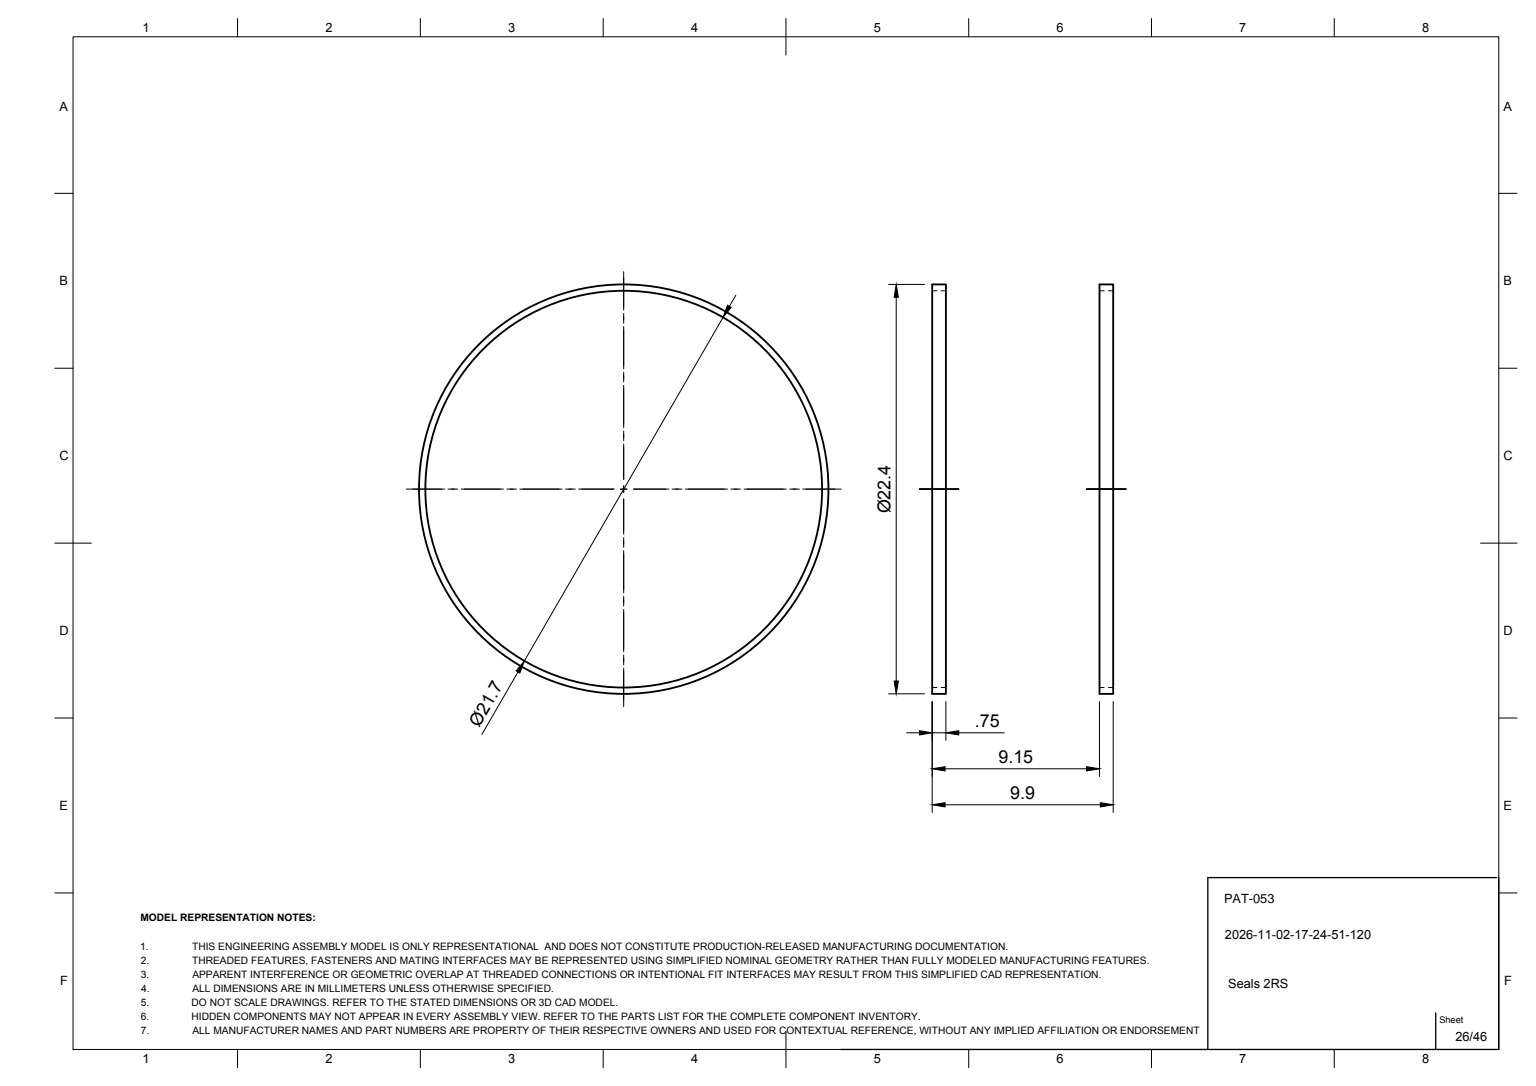
ISO-10303-21;
HEADER;
/* Generated by software containing ST-Developer
 * from STEP Tools, Inc. (www.steptools.com) 
 */

FILE_DESCRIPTION(
/* description */ ('Hand-operated arbor press'),
/* implementation_level */ '2;1');

FILE_NAME(
/* name */ 'Seals 2RS.step',
/* time_stamp */ '2026-10-28T03:25:25-07:00',
/* author */ (''),
/* organization */ (''),
/* preprocessor_version */ 'ST-DEVELOPER v20.2',
/* originating_system */ 'Autodesk Translation Framework v15.17.0.0',
/* authorisation */ '');

FILE_SCHEMA (('AUTOMOTIVE_DESIGN { 1 0 10303 214 3 1 1 }'));
ENDSEC;

DATA;
#10=MECHANICAL_DESIGN_GEOMETRIC_PRESENTATION_REPRESENTATION('',(#612,#613),#32751);
#522=SHAPE_REPRESENTATION_RELATIONSHIP('SRR','None',#32952,#564);
#564=ADVANCED_BREP_SHAPE_REPRESENTATION('',(#660,#661),#32726);
#612=STYLED_ITEM('',(#33242),#660);
#613=STYLED_ITEM('',(#33242),#661);
#660=MANIFOLD_SOLID_BREP('Body1',#12510);
#661=MANIFOLD_SOLID_BREP('Body2',#12511);
#807=FACE_BOUND('',#2361,.T.);
#808=FACE_BOUND('',#2364,.T.);
#809=FACE_BOUND('',#2367,.T.);
#810=FACE_BOUND('',#2370,.T.);
#989=PLANE('',#13521);
#990=PLANE('',#13526);
#991=PLANE('',#13529);
#992=PLANE('',#13534);
#1552=FACE_OUTER_BOUND('',#2360,.T.);
#1553=FACE_OUTER_BOUND('',#2362,.T.);
#1554=FACE_OUTER_BOUND('',#2363,.T.);
#1555=FACE_OUTER_BOUND('',#2365,.T.);
#1556=FACE_OUTER_BOUND('',#2366,.T.);
#1557=FACE_OUTER_BOUND('',#2368,.T.);
#1558=FACE_OUTER_BOUND('',#2369,.T.);
#1559=FACE_OUTER_BOUND('',#2371,.T.);
#2360=EDGE_LOOP('',(#9516));
#2361=EDGE_LOOP('',(#9517));
#2362=EDGE_LOOP('',(#9518,#9519,#9520,#9521));
#2363=EDGE_LOOP('',(#9522));
#2364=EDGE_LOOP('',(#9523));
#2365=EDGE_LOOP('',(#9524,#9525,#9526,#9527));
#2366=EDGE_LOOP('',(#9528));
#2367=EDGE_LOOP('',(#9529));
#2368=EDGE_LOOP('',(#9530,#9531,#9532,#9533));
#2369=EDGE_LOOP('',(#9534));
#2370=EDGE_LOOP('',(#9535));
#2371=EDGE_LOOP('',(#9536,#9537,#9538,#9539));
#3167=LINE('',#19223,#4338);
#3168=LINE('',#19228,#4339);
#3169=LINE('',#19237,#4340);
#3170=LINE('',#19242,#4341);
#4338=VECTOR('',#15552,1.119765);
#4339=VECTOR('',#15559,1.085235);
#4340=VECTOR('',#15570,1.119765);
#4341=VECTOR('',#15577,1.085235);
#5405=CIRCLE('',#13522,1.119765);
#5406=CIRCLE('',#13523,1.085235);
#5407=CIRCLE('',#13525,1.119765);
#5408=CIRCLE('',#13527,1.085235);
#5409=CIRCLE('',#13530,1.119765);
#5410=CIRCLE('',#13531,1.085235);
#5411=CIRCLE('',#13533,1.119765);
#5412=CIRCLE('',#13535,1.085235);
#5960=VERTEX_POINT('',#19216);
#5961=VERTEX_POINT('',#19218);
#5962=VERTEX_POINT('',#19221);
#5963=VERTEX_POINT('',#19225);
#5964=VERTEX_POINT('',#19230);
#5965=VERTEX_POINT('',#19232);
#5966=VERTEX_POINT('',#19235);
#5967=VERTEX_POINT('',#19239);
#7261=EDGE_CURVE('',#5960,#5960,#5405,.T.);
#7262=EDGE_CURVE('',#5961,#5961,#5406,.T.);
#7263=EDGE_CURVE('',#5962,#5962,#5407,.T.);
#7264=EDGE_CURVE('',#5962,#5960,#3167,.T.);
#7265=EDGE_CURVE('',#5963,#5963,#5408,.T.);
#7266=EDGE_CURVE('',#5963,#5961,#3168,.T.);
#7267=EDGE_CURVE('',#5964,#5964,#5409,.T.);
#7268=EDGE_CURVE('',#5965,#5965,#5410,.T.);
#7269=EDGE_CURVE('',#5966,#5966,#5411,.T.);
#7270=EDGE_CURVE('',#5966,#5964,#3169,.T.);
#7271=EDGE_CURVE('',#5967,#5967,#5412,.T.);
#7272=EDGE_CURVE('',#5967,#5965,#3170,.T.);
#9516=ORIENTED_EDGE('',*,*,#7261,.F.);
#9517=ORIENTED_EDGE('',*,*,#7262,.T.);
#9518=ORIENTED_EDGE('',*,*,#7263,.F.);
#9519=ORIENTED_EDGE('',*,*,#7264,.T.);
#9520=ORIENTED_EDGE('',*,*,#7261,.T.);
#9521=ORIENTED_EDGE('',*,*,#7264,.F.);
#9522=ORIENTED_EDGE('',*,*,#7263,.T.);
#9523=ORIENTED_EDGE('',*,*,#7265,.F.);
#9524=ORIENTED_EDGE('',*,*,#7265,.T.);
#9525=ORIENTED_EDGE('',*,*,#7266,.T.);
#9526=ORIENTED_EDGE('',*,*,#7262,.F.);
#9527=ORIENTED_EDGE('',*,*,#7266,.F.);
#9528=ORIENTED_EDGE('',*,*,#7267,.F.);
#9529=ORIENTED_EDGE('',*,*,#7268,.T.);
#9530=ORIENTED_EDGE('',*,*,#7269,.F.);
#9531=ORIENTED_EDGE('',*,*,#7270,.T.);
#9532=ORIENTED_EDGE('',*,*,#7267,.T.);
#9533=ORIENTED_EDGE('',*,*,#7270,.F.);
#9534=ORIENTED_EDGE('',*,*,#7269,.T.);
#9535=ORIENTED_EDGE('',*,*,#7271,.F.);
#9536=ORIENTED_EDGE('',*,*,#7271,.T.);
#9537=ORIENTED_EDGE('',*,*,#7272,.T.);
#9538=ORIENTED_EDGE('',*,*,#7268,.F.);
#9539=ORIENTED_EDGE('',*,*,#7272,.F.);
#11737=CYLINDRICAL_SURFACE('',#13524,1.119765);
#11738=CYLINDRICAL_SURFACE('',#13528,1.085235);
#11739=CYLINDRICAL_SURFACE('',#13532,1.119765);
#11740=CYLINDRICAL_SURFACE('',#13536,1.085235);
#12061=ADVANCED_FACE('',(#1552,#807),#989,.T.);
#12062=ADVANCED_FACE('',(#1553),#11737,.T.);
#12063=ADVANCED_FACE('',(#1554,#808),#990,.T.);
#12064=ADVANCED_FACE('',(#1555),#11738,.F.);
#12065=ADVANCED_FACE('',(#1556,#809),#991,.T.);
#12066=ADVANCED_FACE('',(#1557),#11739,.T.);
#12067=ADVANCED_FACE('',(#1558,#810),#992,.T.);
#12068=ADVANCED_FACE('',(#1559),#11740,.F.);
#12510=CLOSED_SHELL('',(#12061,#12062,#12063,#12064));
#12511=CLOSED_SHELL('',(#12065,#12066,#12067,#12068));
#13520=AXIS2_PLACEMENT_3D('',#19214,#15540,#15541);
#13521=AXIS2_PLACEMENT_3D('',#19215,#15542,#15543);
#13522=AXIS2_PLACEMENT_3D('',#19217,#15544,#15545);
#13523=AXIS2_PLACEMENT_3D('',#19219,#15546,#15547);
#13524=AXIS2_PLACEMENT_3D('',#19220,#15548,#15549);
#13525=AXIS2_PLACEMENT_3D('',#19222,#15550,#15551);
#13526=AXIS2_PLACEMENT_3D('',#19224,#15553,#15554);
#13527=AXIS2_PLACEMENT_3D('',#19226,#15555,#15556);
#13528=AXIS2_PLACEMENT_3D('',#19227,#15557,#15558);
#13529=AXIS2_PLACEMENT_3D('',#19229,#15560,#15561);
#13530=AXIS2_PLACEMENT_3D('',#19231,#15562,#15563);
#13531=AXIS2_PLACEMENT_3D('',#19233,#15564,#15565);
#13532=AXIS2_PLACEMENT_3D('',#19234,#15566,#15567);
#13533=AXIS2_PLACEMENT_3D('',#19236,#15568,#15569);
#13534=AXIS2_PLACEMENT_3D('',#19238,#15571,#15572);
#13535=AXIS2_PLACEMENT_3D('',#19240,#15573,#15574);
#13536=AXIS2_PLACEMENT_3D('',#19241,#15575,#15576);
#15540=DIRECTION('axis',(0.,0.,1.));
#15541=DIRECTION('refdir',(1.,0.,0.));
#15542=DIRECTION('center_axis',(0.,1.,0.));
#15543=DIRECTION('ref_axis',(0.,0.,1.));
#15544=DIRECTION('center_axis',(0.,-1.,0.));
#15545=DIRECTION('ref_axis',(1.,0.,0.));
#15546=DIRECTION('center_axis',(0.,-1.,0.));
#15547=DIRECTION('ref_axis',(1.,0.,0.));
#15548=DIRECTION('center_axis',(0.,-1.,0.));
#15549=DIRECTION('ref_axis',(1.,0.,0.));
#15550=DIRECTION('center_axis',(0.,-1.,0.));
#15551=DIRECTION('ref_axis',(1.,0.,0.));
#15552=DIRECTION('',(0.,1.,0.));
#15553=DIRECTION('center_axis',(0.,-1.,0.));
#15554=DIRECTION('ref_axis',(0.,0.,-1.));
#15555=DIRECTION('center_axis',(0.,-1.,0.));
#15556=DIRECTION('ref_axis',(1.,0.,0.));
#15557=DIRECTION('center_axis',(0.,-1.,0.));
#15558=DIRECTION('ref_axis',(1.,0.,0.));
#15559=DIRECTION('',(0.,1.,0.));
#15560=DIRECTION('center_axis',(0.,1.,0.));
#15561=DIRECTION('ref_axis',(0.,0.,1.));
#15562=DIRECTION('center_axis',(0.,-1.,0.));
#15563=DIRECTION('ref_axis',(1.,0.,0.));
#15564=DIRECTION('center_axis',(0.,-1.,0.));
#15565=DIRECTION('ref_axis',(1.,0.,0.));
#15566=DIRECTION('center_axis',(0.,-1.,0.));
#15567=DIRECTION('ref_axis',(1.,0.,0.));
#15568=DIRECTION('center_axis',(0.,-1.,0.));
#15569=DIRECTION('ref_axis',(1.,0.,0.));
#15570=DIRECTION('',(0.,1.,0.));
#15571=DIRECTION('center_axis',(0.,-1.,0.));
#15572=DIRECTION('ref_axis',(0.,0.,-1.));
#15573=DIRECTION('center_axis',(0.,-1.,0.));
#15574=DIRECTION('ref_axis',(1.,0.,0.));
#15575=DIRECTION('center_axis',(0.,-1.,0.));
#15576=DIRECTION('ref_axis',(1.,0.,0.));
#15577=DIRECTION('',(0.,1.,0.));
#19214=CARTESIAN_POINT('',(0.,0.,0.));
#19215=CARTESIAN_POINT('Origin',(1.119765,0.495,0.));
#19216=CARTESIAN_POINT('',(-1.119765,0.495,-1.37131662304724E-16));
#19217=CARTESIAN_POINT('Origin',(0.,0.495,0.));
#19218=CARTESIAN_POINT('',(-1.085235,0.495,-1.32902956907268E-16));
#19219=CARTESIAN_POINT('Origin',(0.,0.495,0.));
#19220=CARTESIAN_POINT('Origin',(0.,0.4575,0.));
#19221=CARTESIAN_POINT('',(-1.119765,0.42,-1.37131662304724E-16));
#19222=CARTESIAN_POINT('Origin',(0.,0.42,0.));
#19223=CARTESIAN_POINT('',(-1.119765,0.4575,-1.37131662304724E-16));
#19224=CARTESIAN_POINT('Origin',(1.085235,0.42,0.));
#19225=CARTESIAN_POINT('',(-1.085235,0.42,-1.32902956907268E-16));
#19226=CARTESIAN_POINT('Origin',(0.,0.42,0.));
#19227=CARTESIAN_POINT('Origin',(0.,0.4575,0.));
#19228=CARTESIAN_POINT('',(-1.085235,0.4575,-1.32902956907268E-16));
#19229=CARTESIAN_POINT('Origin',(1.119765,-0.42,0.));
#19230=CARTESIAN_POINT('',(-1.119765,-0.42,-1.37131662304724E-16));
#19231=CARTESIAN_POINT('Origin',(0.,-0.42,0.));
#19232=CARTESIAN_POINT('',(-1.085235,-0.42,-1.32902956907268E-16));
#19233=CARTESIAN_POINT('Origin',(0.,-0.42,0.));
#19234=CARTESIAN_POINT('Origin',(0.,-0.4575,0.));
#19235=CARTESIAN_POINT('',(-1.119765,-0.495,-1.37131662304724E-16));
#19236=CARTESIAN_POINT('Origin',(0.,-0.495,0.));
#19237=CARTESIAN_POINT('',(-1.119765,-0.4575,-1.37131662304724E-16));
#19238=CARTESIAN_POINT('Origin',(1.085235,-0.495,0.));
#19239=CARTESIAN_POINT('',(-1.085235,-0.495,-1.32902956907268E-16));
#19240=CARTESIAN_POINT('Origin',(0.,-0.495,0.));
#19241=CARTESIAN_POINT('Origin',(0.,-0.4575,0.));
#19242=CARTESIAN_POINT('',(-1.085235,-0.4575,-1.32902956907268E-16));
#32677=UNCERTAINTY_MEASURE_WITH_UNIT(LENGTH_MEASURE(0.001),#32752,
'DISTANCE_ACCURACY_VALUE',
'Maximum model space distance between geometric entities at asserted c
onnectivities');
#32702=UNCERTAINTY_MEASURE_WITH_UNIT(LENGTH_MEASURE(0.001),#32752,
'DISTANCE_ACCURACY_VALUE',
'Maximum model space distance between geometric entities at asserted c
onnectivities');
#32726=(
GEOMETRIC_REPRESENTATION_CONTEXT(3)
GLOBAL_UNCERTAINTY_ASSIGNED_CONTEXT((#32677))
GLOBAL_UNIT_ASSIGNED_CONTEXT((#32752,#32754,#32755))
REPRESENTATION_CONTEXT('','3D')
);
#32751=(
GEOMETRIC_REPRESENTATION_CONTEXT(3)
GLOBAL_UNCERTAINTY_ASSIGNED_CONTEXT((#32702))
GLOBAL_UNIT_ASSIGNED_CONTEXT((#32752,#32754,#32755))
REPRESENTATION_CONTEXT('','3D')
);
#32752=(
LENGTH_UNIT()
NAMED_UNIT(*)
SI_UNIT(.CENTI.,.METRE.)
);
#32754=(
NAMED_UNIT(*)
PLANE_ANGLE_UNIT()
SI_UNIT($,.RADIAN.)
);
#32755=(
NAMED_UNIT(*)
SI_UNIT($,.STERADIAN.)
SOLID_ANGLE_UNIT()
);
#32779=SHAPE_DEFINITION_REPRESENTATION(#32827,#32952);
#32827=PRODUCT_DEFINITION_SHAPE('',$,#33001);
#32952=SHAPE_REPRESENTATION('',(#13520),#32726);
#32977=PRODUCT_DEFINITION_CONTEXT('part definition',#33123,'design');
#33001=PRODUCT_DEFINITION('Seals 2RS','Seals 2RS',#33049,#32977);
#33049=PRODUCT_DEFINITION_FORMATION('',$,#33148);
#33123=APPLICATION_CONTEXT(
'Core Data for Automotive Mechanical Design Process');
#33124=PRODUCT_CONTEXT('part definition',#33123,'mechanical');
#33148=PRODUCT('Seals 2RS','Seals 2RS','Seals 2RS',(#33124));
#33236=COLOUR_RGB('Grey',0.48,0.52,0.57);
#33237=FILL_AREA_STYLE_COLOUR('',#33236);
#33238=FILL_AREA_STYLE('',(#33237));
#33239=SURFACE_STYLE_FILL_AREA(#33238);
#33240=SURFACE_SIDE_STYLE('',(#33239));
#33241=SURFACE_STYLE_USAGE(.BOTH.,#33240);
#33242=PRESENTATION_STYLE_ASSIGNMENT((#33241));
ENDSEC;
END-ISO-10303-21;
